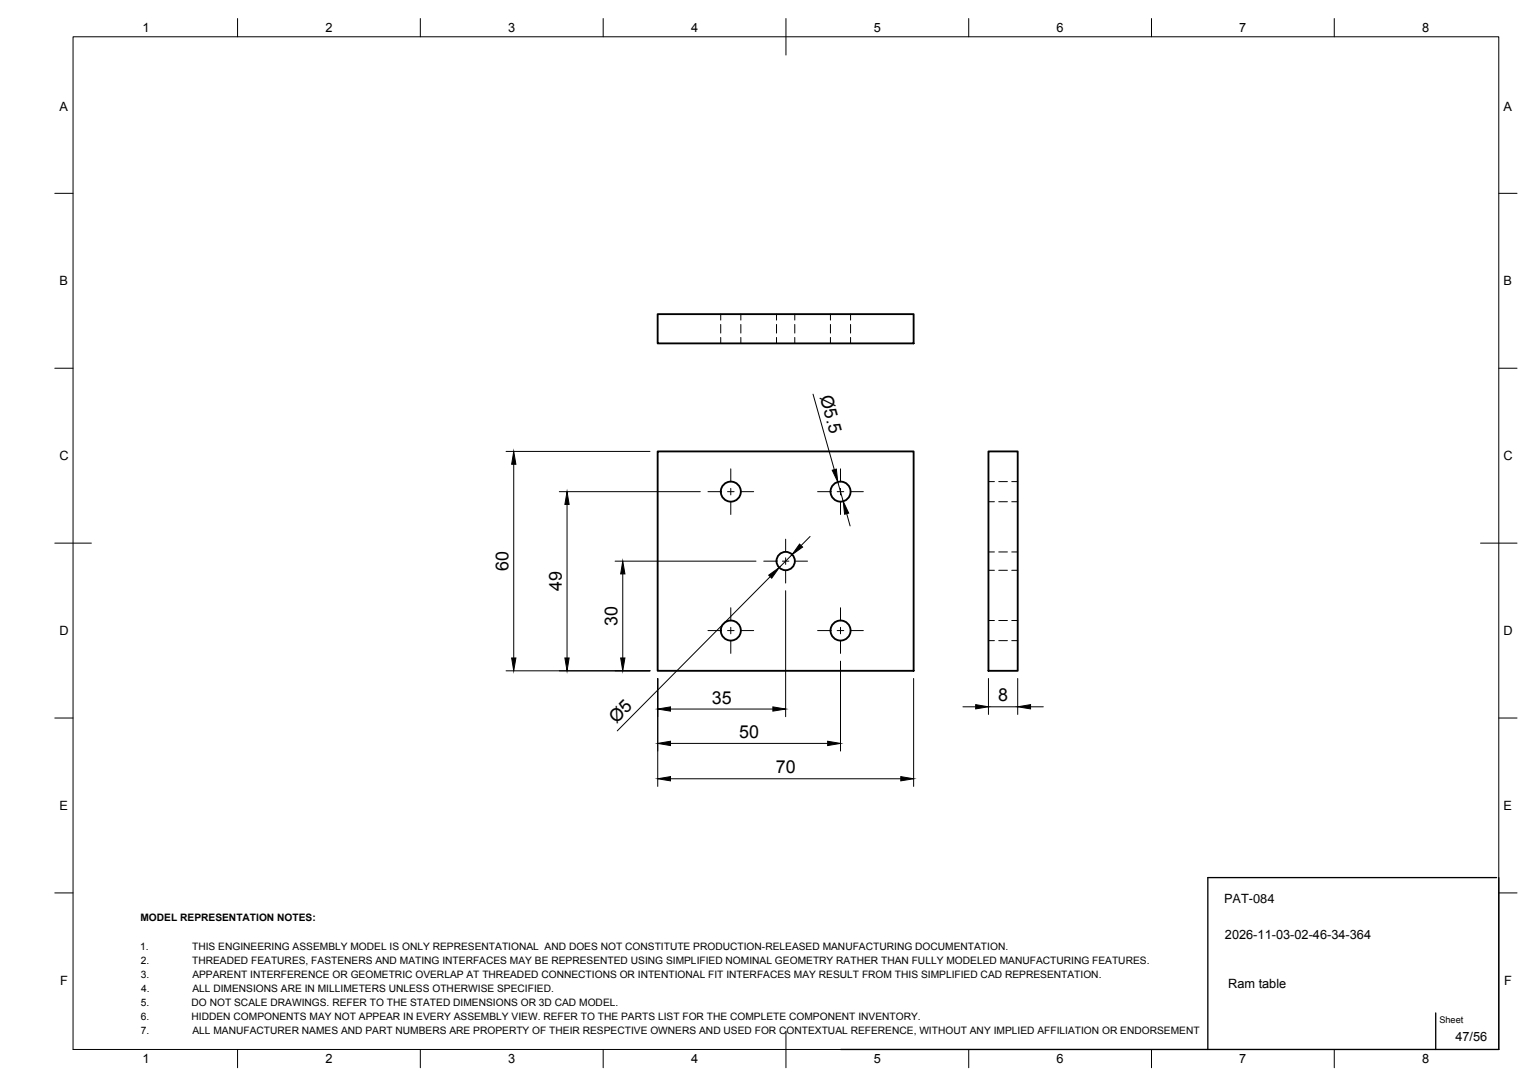
ISO-10303-21;
HEADER;
/* Generated by software containing ST-Developer
 * from STEP Tools, Inc. (www.steptools.com) 
 */

FILE_DESCRIPTION(
/* description */ ('Quick-return (Whitworth) mechanism'),
/* implementation_level */ '2;1');

FILE_NAME(
/* name */ 'Ram table.step',
/* time_stamp */ '2026-10-28T03:25:57-07:00',
/* author */ (''),
/* organization */ (''),
/* preprocessor_version */ 'ST-DEVELOPER v20.2',
/* originating_system */ 'Autodesk Translation Framework v15.17.0.0',
/* authorisation */ '');

FILE_SCHEMA (('AUTOMOTIVE_DESIGN { 1 0 10303 214 3 1 1 }'));
ENDSEC;

DATA;
#10=MECHANICAL_DESIGN_GEOMETRIC_PRESENTATION_REPRESENTATION('',(#532),#14878);
#436=SHAPE_REPRESENTATION_RELATIONSHIP('SRR','None',#15110,#480);
#480=ADVANCED_BREP_SHAPE_REPRESENTATION('',(#583),#14867);
#532=STYLED_ITEM('',(#15420),#583);
#583=MANIFOLD_SOLID_BREP('Body1',#7887);
#757=FACE_BOUND('',#2049,.T.);
#758=FACE_BOUND('',#2050,.T.);
#759=FACE_BOUND('',#2051,.T.);
#760=FACE_BOUND('',#2052,.T.);
#761=FACE_BOUND('',#2053,.T.);
#762=FACE_BOUND('',#2055,.T.);
#763=FACE_BOUND('',#2056,.T.);
#764=FACE_BOUND('',#2057,.T.);
#765=FACE_BOUND('',#2058,.T.);
#766=FACE_BOUND('',#2059,.T.);
#970=PLANE('',#9166);
#971=PLANE('',#9167);
#972=PLANE('',#9168);
#973=PLANE('',#9169);
#974=PLANE('',#9170);
#975=PLANE('',#9171);
#1407=FACE_OUTER_BOUND('',#2039,.T.);
#1408=FACE_OUTER_BOUND('',#2040,.T.);
#1409=FACE_OUTER_BOUND('',#2041,.T.);
#1410=FACE_OUTER_BOUND('',#2042,.T.);
#1411=FACE_OUTER_BOUND('',#2043,.T.);
#1412=FACE_OUTER_BOUND('',#2044,.T.);
#1413=FACE_OUTER_BOUND('',#2045,.T.);
#1414=FACE_OUTER_BOUND('',#2046,.T.);
#1415=FACE_OUTER_BOUND('',#2047,.T.);
#1416=FACE_OUTER_BOUND('',#2048,.T.);
#1417=FACE_OUTER_BOUND('',#2054,.T.);
#2039=EDGE_LOOP('',(#6736,#6737,#6738,#6739));
#2040=EDGE_LOOP('',(#6740,#6741,#6742,#6743));
#2041=EDGE_LOOP('',(#6744,#6745,#6746,#6747));
#2042=EDGE_LOOP('',(#6748,#6749,#6750,#6751));
#2043=EDGE_LOOP('',(#6752,#6753,#6754,#6755));
#2044=EDGE_LOOP('',(#6756,#6757,#6758,#6759));
#2045=EDGE_LOOP('',(#6760,#6761,#6762,#6763));
#2046=EDGE_LOOP('',(#6764,#6765,#6766,#6767));
#2047=EDGE_LOOP('',(#6768,#6769,#6770,#6771));
#2048=EDGE_LOOP('',(#6772,#6773,#6774,#6775));
#2049=EDGE_LOOP('',(#6776));
#2050=EDGE_LOOP('',(#6777));
#2051=EDGE_LOOP('',(#6778));
#2052=EDGE_LOOP('',(#6779));
#2053=EDGE_LOOP('',(#6780));
#2054=EDGE_LOOP('',(#6781,#6782,#6783,#6784));
#2055=EDGE_LOOP('',(#6785));
#2056=EDGE_LOOP('',(#6786));
#2057=EDGE_LOOP('',(#6787));
#2058=EDGE_LOOP('',(#6788));
#2059=EDGE_LOOP('',(#6789));
#2516=LINE('',#14196,#3039);
#2517=LINE('',#14202,#3040);
#2518=LINE('',#14208,#3041);
#2519=LINE('',#14214,#3042);
#2520=LINE('',#14220,#3043);
#2521=LINE('',#14225,#3044);
#2522=LINE('',#14227,#3045);
#2523=LINE('',#14229,#3046);
#2524=LINE('',#14230,#3047);
#2525=LINE('',#14233,#3048);
#2526=LINE('',#14235,#3049);
#2527=LINE('',#14236,#3050);
#2528=LINE('',#14239,#3051);
#2529=LINE('',#14241,#3052);
#2530=LINE('',#14242,#3053);
#2531=LINE('',#14244,#3054);
#2532=LINE('',#14245,#3055);
#3039=VECTOR('',#11281,0.25);
#3040=VECTOR('',#11288,0.275);
#3041=VECTOR('',#11295,0.275);
#3042=VECTOR('',#11302,0.275);
#3043=VECTOR('',#11309,0.275);
#3044=VECTOR('',#11314,1.);
#3045=VECTOR('',#11315,1.);
#3046=VECTOR('',#11316,1.);
#3047=VECTOR('',#11317,1.);
#3048=VECTOR('',#11320,1.);
#3049=VECTOR('',#11321,1.);
#3050=VECTOR('',#11322,1.);
#3051=VECTOR('',#11325,1.);
#3052=VECTOR('',#11326,1.);
#3053=VECTOR('',#11327,1.);
#3054=VECTOR('',#11330,1.);
#3055=VECTOR('',#11331,1.);
#3571=CIRCLE('',#9152,0.25);
#3572=CIRCLE('',#9153,0.25);
#3573=CIRCLE('',#9155,0.275);
#3574=CIRCLE('',#9156,0.275);
#3575=CIRCLE('',#9158,0.275);
#3576=CIRCLE('',#9159,0.275);
#3577=CIRCLE('',#9161,0.275);
#3578=CIRCLE('',#9162,0.275);
#3579=CIRCLE('',#9164,0.275);
#3580=CIRCLE('',#9165,0.275);
#4132=VERTEX_POINT('',#14193);
#4133=VERTEX_POINT('',#14195);
#4134=VERTEX_POINT('',#14199);
#4135=VERTEX_POINT('',#14201);
#4136=VERTEX_POINT('',#14205);
#4137=VERTEX_POINT('',#14207);
#4138=VERTEX_POINT('',#14211);
#4139=VERTEX_POINT('',#14213);
#4140=VERTEX_POINT('',#14217);
#4141=VERTEX_POINT('',#14219);
#4142=VERTEX_POINT('',#14223);
#4143=VERTEX_POINT('',#14224);
#4144=VERTEX_POINT('',#14226);
#4145=VERTEX_POINT('',#14228);
#4146=VERTEX_POINT('',#14232);
#4147=VERTEX_POINT('',#14234);
#4148=VERTEX_POINT('',#14238);
#4149=VERTEX_POINT('',#14240);
#5025=EDGE_CURVE('',#4132,#4132,#3571,.T.);
#5026=EDGE_CURVE('',#4132,#4133,#2516,.T.);
#5027=EDGE_CURVE('',#4133,#4133,#3572,.T.);
#5028=EDGE_CURVE('',#4134,#4134,#3573,.T.);
#5029=EDGE_CURVE('',#4134,#4135,#2517,.T.);
#5030=EDGE_CURVE('',#4135,#4135,#3574,.T.);
#5031=EDGE_CURVE('',#4136,#4136,#3575,.T.);
#5032=EDGE_CURVE('',#4136,#4137,#2518,.T.);
#5033=EDGE_CURVE('',#4137,#4137,#3576,.T.);
#5034=EDGE_CURVE('',#4138,#4138,#3577,.T.);
#5035=EDGE_CURVE('',#4138,#4139,#2519,.T.);
#5036=EDGE_CURVE('',#4139,#4139,#3578,.T.);
#5037=EDGE_CURVE('',#4140,#4140,#3579,.T.);
#5038=EDGE_CURVE('',#4140,#4141,#2520,.T.);
#5039=EDGE_CURVE('',#4141,#4141,#3580,.T.);
#5040=EDGE_CURVE('',#4142,#4143,#2521,.T.);
#5041=EDGE_CURVE('',#4143,#4144,#2522,.T.);
#5042=EDGE_CURVE('',#4145,#4144,#2523,.T.);
#5043=EDGE_CURVE('',#4142,#4145,#2524,.T.);
#5044=EDGE_CURVE('',#4146,#4142,#2525,.T.);
#5045=EDGE_CURVE('',#4147,#4145,#2526,.T.);
#5046=EDGE_CURVE('',#4146,#4147,#2527,.T.);
#5047=EDGE_CURVE('',#4148,#4146,#2528,.T.);
#5048=EDGE_CURVE('',#4149,#4147,#2529,.T.);
#5049=EDGE_CURVE('',#4148,#4149,#2530,.T.);
#5050=EDGE_CURVE('',#4143,#4148,#2531,.T.);
#5051=EDGE_CURVE('',#4144,#4149,#2532,.T.);
#6736=ORIENTED_EDGE('',*,*,#5025,.F.);
#6737=ORIENTED_EDGE('',*,*,#5026,.T.);
#6738=ORIENTED_EDGE('',*,*,#5027,.F.);
#6739=ORIENTED_EDGE('',*,*,#5026,.F.);
#6740=ORIENTED_EDGE('',*,*,#5028,.F.);
#6741=ORIENTED_EDGE('',*,*,#5029,.T.);
#6742=ORIENTED_EDGE('',*,*,#5030,.F.);
#6743=ORIENTED_EDGE('',*,*,#5029,.F.);
#6744=ORIENTED_EDGE('',*,*,#5031,.F.);
#6745=ORIENTED_EDGE('',*,*,#5032,.T.);
#6746=ORIENTED_EDGE('',*,*,#5033,.F.);
#6747=ORIENTED_EDGE('',*,*,#5032,.F.);
#6748=ORIENTED_EDGE('',*,*,#5034,.F.);
#6749=ORIENTED_EDGE('',*,*,#5035,.T.);
#6750=ORIENTED_EDGE('',*,*,#5036,.F.);
#6751=ORIENTED_EDGE('',*,*,#5035,.F.);
#6752=ORIENTED_EDGE('',*,*,#5037,.F.);
#6753=ORIENTED_EDGE('',*,*,#5038,.T.);
#6754=ORIENTED_EDGE('',*,*,#5039,.F.);
#6755=ORIENTED_EDGE('',*,*,#5038,.F.);
#6756=ORIENTED_EDGE('',*,*,#5040,.T.);
#6757=ORIENTED_EDGE('',*,*,#5041,.T.);
#6758=ORIENTED_EDGE('',*,*,#5042,.F.);
#6759=ORIENTED_EDGE('',*,*,#5043,.F.);
#6760=ORIENTED_EDGE('',*,*,#5044,.T.);
#6761=ORIENTED_EDGE('',*,*,#5043,.T.);
#6762=ORIENTED_EDGE('',*,*,#5045,.F.);
#6763=ORIENTED_EDGE('',*,*,#5046,.F.);
#6764=ORIENTED_EDGE('',*,*,#5047,.T.);
#6765=ORIENTED_EDGE('',*,*,#5046,.T.);
#6766=ORIENTED_EDGE('',*,*,#5048,.F.);
#6767=ORIENTED_EDGE('',*,*,#5049,.F.);
#6768=ORIENTED_EDGE('',*,*,#5050,.T.);
#6769=ORIENTED_EDGE('',*,*,#5049,.T.);
#6770=ORIENTED_EDGE('',*,*,#5051,.F.);
#6771=ORIENTED_EDGE('',*,*,#5041,.F.);
#6772=ORIENTED_EDGE('',*,*,#5051,.T.);
#6773=ORIENTED_EDGE('',*,*,#5048,.T.);
#6774=ORIENTED_EDGE('',*,*,#5045,.T.);
#6775=ORIENTED_EDGE('',*,*,#5042,.T.);
#6776=ORIENTED_EDGE('',*,*,#5027,.T.);
#6777=ORIENTED_EDGE('',*,*,#5030,.T.);
#6778=ORIENTED_EDGE('',*,*,#5033,.T.);
#6779=ORIENTED_EDGE('',*,*,#5036,.T.);
#6780=ORIENTED_EDGE('',*,*,#5039,.T.);
#6781=ORIENTED_EDGE('',*,*,#5050,.F.);
#6782=ORIENTED_EDGE('',*,*,#5040,.F.);
#6783=ORIENTED_EDGE('',*,*,#5044,.F.);
#6784=ORIENTED_EDGE('',*,*,#5047,.F.);
#6785=ORIENTED_EDGE('',*,*,#5025,.T.);
#6786=ORIENTED_EDGE('',*,*,#5028,.T.);
#6787=ORIENTED_EDGE('',*,*,#5031,.T.);
#6788=ORIENTED_EDGE('',*,*,#5034,.T.);
#6789=ORIENTED_EDGE('',*,*,#5037,.T.);
#7355=CYLINDRICAL_SURFACE('',#9151,0.25);
#7356=CYLINDRICAL_SURFACE('',#9154,0.275);
#7357=CYLINDRICAL_SURFACE('',#9157,0.275);
#7358=CYLINDRICAL_SURFACE('',#9160,0.275);
#7359=CYLINDRICAL_SURFACE('',#9163,0.275);
#7738=ADVANCED_FACE('',(#1407),#7355,.F.);
#7739=ADVANCED_FACE('',(#1408),#7356,.F.);
#7740=ADVANCED_FACE('',(#1409),#7357,.F.);
#7741=ADVANCED_FACE('',(#1410),#7358,.F.);
#7742=ADVANCED_FACE('',(#1411),#7359,.F.);
#7743=ADVANCED_FACE('',(#1412),#970,.T.);
#7744=ADVANCED_FACE('',(#1413),#971,.T.);
#7745=ADVANCED_FACE('',(#1414),#972,.T.);
#7746=ADVANCED_FACE('',(#1415),#973,.T.);
#7747=ADVANCED_FACE('',(#1416,#757,#758,#759,#760,#761),#974,.T.);
#7748=ADVANCED_FACE('',(#1417,#762,#763,#764,#765,#766),#975,.F.);
#7887=CLOSED_SHELL('',(#7738,#7739,#7740,#7741,#7742,#7743,#7744,#7745,
#7746,#7747,#7748));
#9150=AXIS2_PLACEMENT_3D('',#14191,#11275,#11276);
#9151=AXIS2_PLACEMENT_3D('',#14192,#11277,#11278);
#9152=AXIS2_PLACEMENT_3D('',#14194,#11279,#11280);
#9153=AXIS2_PLACEMENT_3D('',#14197,#11282,#11283);
#9154=AXIS2_PLACEMENT_3D('',#14198,#11284,#11285);
#9155=AXIS2_PLACEMENT_3D('',#14200,#11286,#11287);
#9156=AXIS2_PLACEMENT_3D('',#14203,#11289,#11290);
#9157=AXIS2_PLACEMENT_3D('',#14204,#11291,#11292);
#9158=AXIS2_PLACEMENT_3D('',#14206,#11293,#11294);
#9159=AXIS2_PLACEMENT_3D('',#14209,#11296,#11297);
#9160=AXIS2_PLACEMENT_3D('',#14210,#11298,#11299);
#9161=AXIS2_PLACEMENT_3D('',#14212,#11300,#11301);
#9162=AXIS2_PLACEMENT_3D('',#14215,#11303,#11304);
#9163=AXIS2_PLACEMENT_3D('',#14216,#11305,#11306);
#9164=AXIS2_PLACEMENT_3D('',#14218,#11307,#11308);
#9165=AXIS2_PLACEMENT_3D('',#14221,#11310,#11311);
#9166=AXIS2_PLACEMENT_3D('',#14222,#11312,#11313);
#9167=AXIS2_PLACEMENT_3D('',#14231,#11318,#11319);
#9168=AXIS2_PLACEMENT_3D('',#14237,#11323,#11324);
#9169=AXIS2_PLACEMENT_3D('',#14243,#11328,#11329);
#9170=AXIS2_PLACEMENT_3D('',#14246,#11332,#11333);
#9171=AXIS2_PLACEMENT_3D('',#14247,#11334,#11335);
#11275=DIRECTION('axis',(0.,0.,1.));
#11276=DIRECTION('refdir',(1.,0.,0.));
#11277=DIRECTION('center_axis',(0.,0.,1.));
#11278=DIRECTION('ref_axis',(1.,0.,0.));
#11279=DIRECTION('center_axis',(0.,0.,1.));
#11280=DIRECTION('ref_axis',(1.,0.,0.));
#11281=DIRECTION('',(0.,0.,1.));
#11282=DIRECTION('center_axis',(0.,0.,-1.));
#11283=DIRECTION('ref_axis',(1.,0.,0.));
#11284=DIRECTION('center_axis',(0.,0.,1.));
#11285=DIRECTION('ref_axis',(1.,0.,0.));
#11286=DIRECTION('center_axis',(0.,0.,1.));
#11287=DIRECTION('ref_axis',(1.,0.,0.));
#11288=DIRECTION('',(0.,0.,1.));
#11289=DIRECTION('center_axis',(0.,0.,-1.));
#11290=DIRECTION('ref_axis',(1.,0.,0.));
#11291=DIRECTION('center_axis',(0.,0.,1.));
#11292=DIRECTION('ref_axis',(1.,0.,0.));
#11293=DIRECTION('center_axis',(0.,0.,1.));
#11294=DIRECTION('ref_axis',(1.,0.,0.));
#11295=DIRECTION('',(0.,0.,1.));
#11296=DIRECTION('center_axis',(0.,0.,-1.));
#11297=DIRECTION('ref_axis',(1.,0.,0.));
#11298=DIRECTION('center_axis',(0.,0.,1.));
#11299=DIRECTION('ref_axis',(1.,0.,0.));
#11300=DIRECTION('center_axis',(0.,0.,1.));
#11301=DIRECTION('ref_axis',(1.,0.,0.));
#11302=DIRECTION('',(0.,0.,1.));
#11303=DIRECTION('center_axis',(0.,0.,-1.));
#11304=DIRECTION('ref_axis',(1.,0.,0.));
#11305=DIRECTION('center_axis',(0.,0.,1.));
#11306=DIRECTION('ref_axis',(1.,0.,0.));
#11307=DIRECTION('center_axis',(0.,0.,1.));
#11308=DIRECTION('ref_axis',(1.,0.,0.));
#11309=DIRECTION('',(0.,0.,1.));
#11310=DIRECTION('center_axis',(0.,0.,-1.));
#11311=DIRECTION('ref_axis',(1.,0.,0.));
#11312=DIRECTION('center_axis',(0.,1.,0.));
#11313=DIRECTION('ref_axis',(-1.,0.,0.));
#11314=DIRECTION('',(-1.,0.,0.));
#11315=DIRECTION('',(0.,0.,1.));
#11316=DIRECTION('',(-1.,0.,0.));
#11317=DIRECTION('',(0.,0.,1.));
#11318=DIRECTION('center_axis',(1.,0.,0.));
#11319=DIRECTION('ref_axis',(0.,1.,0.));
#11320=DIRECTION('',(0.,1.,0.));
#11321=DIRECTION('',(0.,1.,0.));
#11322=DIRECTION('',(0.,0.,1.));
#11323=DIRECTION('center_axis',(0.,-1.,0.));
#11324=DIRECTION('ref_axis',(1.,0.,0.));
#11325=DIRECTION('',(1.,0.,0.));
#11326=DIRECTION('',(1.,0.,0.));
#11327=DIRECTION('',(0.,0.,1.));
#11328=DIRECTION('center_axis',(-1.,0.,0.));
#11329=DIRECTION('ref_axis',(0.,-1.,0.));
#11330=DIRECTION('',(0.,-1.,0.));
#11331=DIRECTION('',(0.,-1.,0.));
#11332=DIRECTION('center_axis',(0.,0.,1.));
#11333=DIRECTION('ref_axis',(1.,0.,0.));
#11334=DIRECTION('center_axis',(0.,0.,1.));
#11335=DIRECTION('ref_axis',(1.,0.,0.));
#14191=CARTESIAN_POINT('',(0.,0.,0.));
#14192=CARTESIAN_POINT('Origin',(9.16515138991168,16.,3.3));
#14193=CARTESIAN_POINT('',(8.91515138991168,16.,3.4));
#14194=CARTESIAN_POINT('Origin',(9.16515138991168,16.,3.4));
#14195=CARTESIAN_POINT('',(8.91515138991168,16.,4.2));
#14196=CARTESIAN_POINT('',(8.91515138991168,16.,3.3));
#14197=CARTESIAN_POINT('Origin',(9.16515138991168,16.,4.2));
#14198=CARTESIAN_POINT('Origin',(10.6651513899117,14.1,3.3));
#14199=CARTESIAN_POINT('',(10.3901513899117,14.1,3.4));
#14200=CARTESIAN_POINT('Origin',(10.6651513899117,14.1,3.4));
#14201=CARTESIAN_POINT('',(10.3901513899117,14.1,4.2));
#14202=CARTESIAN_POINT('',(10.3901513899117,14.1,3.3));
#14203=CARTESIAN_POINT('Origin',(10.6651513899117,14.1,4.2));
#14204=CARTESIAN_POINT('Origin',(7.66515138991168,17.9,3.3));
#14205=CARTESIAN_POINT('',(7.39015138991168,17.9,3.4));
#14206=CARTESIAN_POINT('Origin',(7.66515138991168,17.9,3.4));
#14207=CARTESIAN_POINT('',(7.39015138991168,17.9,4.2));
#14208=CARTESIAN_POINT('',(7.39015138991168,17.9,3.3));
#14209=CARTESIAN_POINT('Origin',(7.66515138991168,17.9,4.2));
#14210=CARTESIAN_POINT('Origin',(7.66515138991168,14.1,3.3));
#14211=CARTESIAN_POINT('',(7.39015138991168,14.1,3.4));
#14212=CARTESIAN_POINT('Origin',(7.66515138991168,14.1,3.4));
#14213=CARTESIAN_POINT('',(7.39015138991168,14.1,4.2));
#14214=CARTESIAN_POINT('',(7.39015138991168,14.1,3.3));
#14215=CARTESIAN_POINT('Origin',(7.66515138991168,14.1,4.2));
#14216=CARTESIAN_POINT('Origin',(10.6651513899117,17.9,3.3));
#14217=CARTESIAN_POINT('',(10.3901513899117,17.9,3.4));
#14218=CARTESIAN_POINT('Origin',(10.6651513899117,17.9,3.4));
#14219=CARTESIAN_POINT('',(10.3901513899117,17.9,4.2));
#14220=CARTESIAN_POINT('',(10.3901513899117,17.9,3.3));
#14221=CARTESIAN_POINT('Origin',(10.6651513899117,17.9,4.2));
#14222=CARTESIAN_POINT('Origin',(12.6651513899117,19.,3.4));
#14223=CARTESIAN_POINT('',(12.6651513899117,19.,3.4));
#14224=CARTESIAN_POINT('',(5.66515138991168,19.,3.4));
#14225=CARTESIAN_POINT('',(12.6651513899117,19.,3.4));
#14226=CARTESIAN_POINT('',(5.66515138991168,19.,4.2));
#14227=CARTESIAN_POINT('',(5.66515138991168,19.,3.4));
#14228=CARTESIAN_POINT('',(12.6651513899117,19.,4.2));
#14229=CARTESIAN_POINT('',(12.6651513899117,19.,4.2));
#14230=CARTESIAN_POINT('',(12.6651513899117,19.,3.4));
#14231=CARTESIAN_POINT('Origin',(12.6651513899117,13.,3.4));
#14232=CARTESIAN_POINT('',(12.6651513899117,13.,3.4));
#14233=CARTESIAN_POINT('',(12.6651513899117,13.,3.4));
#14234=CARTESIAN_POINT('',(12.6651513899117,13.,4.2));
#14235=CARTESIAN_POINT('',(12.6651513899117,13.,4.2));
#14236=CARTESIAN_POINT('',(12.6651513899117,13.,3.4));
#14237=CARTESIAN_POINT('Origin',(5.66515138991168,13.,3.4));
#14238=CARTESIAN_POINT('',(5.66515138991168,13.,3.4));
#14239=CARTESIAN_POINT('',(5.66515138991168,13.,3.4));
#14240=CARTESIAN_POINT('',(5.66515138991168,13.,4.2));
#14241=CARTESIAN_POINT('',(5.66515138991168,13.,4.2));
#14242=CARTESIAN_POINT('',(5.66515138991168,13.,3.4));
#14243=CARTESIAN_POINT('Origin',(5.66515138991168,19.,3.4));
#14244=CARTESIAN_POINT('',(5.66515138991168,19.,3.4));
#14245=CARTESIAN_POINT('',(5.66515138991168,19.,4.2));
#14246=CARTESIAN_POINT('Origin',(9.16515138991168,16.,4.2));
#14247=CARTESIAN_POINT('Origin',(9.16515138991168,16.,3.4));
#14813=UNCERTAINTY_MEASURE_WITH_UNIT(LENGTH_MEASURE(0.001),#14879,
'DISTANCE_ACCURACY_VALUE',
'Maximum model space distance between geometric entities at asserted c
onnectivities');
#14824=UNCERTAINTY_MEASURE_WITH_UNIT(LENGTH_MEASURE(0.001),#14879,
'DISTANCE_ACCURACY_VALUE',
'Maximum model space distance between geometric entities at asserted c
onnectivities');
#14867=(
GEOMETRIC_REPRESENTATION_CONTEXT(3)
GLOBAL_UNCERTAINTY_ASSIGNED_CONTEXT((#14813))
GLOBAL_UNIT_ASSIGNED_CONTEXT((#14879,#14881,#14882))
REPRESENTATION_CONTEXT('','3D')
);
#14878=(
GEOMETRIC_REPRESENTATION_CONTEXT(3)
GLOBAL_UNCERTAINTY_ASSIGNED_CONTEXT((#14824))
GLOBAL_UNIT_ASSIGNED_CONTEXT((#14879,#14881,#14882))
REPRESENTATION_CONTEXT('','3D')
);
#14879=(
LENGTH_UNIT()
NAMED_UNIT(*)
SI_UNIT(.CENTI.,.METRE.)
);
#14881=(
NAMED_UNIT(*)
PLANE_ANGLE_UNIT()
SI_UNIT($,.RADIAN.)
);
#14882=(
NAMED_UNIT(*)
SI_UNIT($,.STERADIAN.)
SOLID_ANGLE_UNIT()
);
#14925=SHAPE_DEFINITION_REPRESENTATION(#14987,#15110);
#14987=PRODUCT_DEFINITION_SHAPE('',$,#15164);
#15110=SHAPE_REPRESENTATION('',(#9150),#14867);
#15121=PRODUCT_DEFINITION_CONTEXT('part definition',#15282,'design');
#15164=PRODUCT_DEFINITION('Ram table','Ram table',#15217,#15121);
#15217=PRODUCT_DEFINITION_FORMATION('',$,#15326);
#15282=APPLICATION_CONTEXT(
'Core Data for Automotive Mechanical Design Process');
#15283=PRODUCT_CONTEXT('part definition',#15282,'mechanical');
#15326=PRODUCT('Ram table','Ram table','Ram table',(#15283));
#15414=COLOUR_RGB('Off White',0.89,0.88,0.83);
#15415=FILL_AREA_STYLE_COLOUR('',#15414);
#15416=FILL_AREA_STYLE('',(#15415));
#15417=SURFACE_STYLE_FILL_AREA(#15416);
#15418=SURFACE_SIDE_STYLE('',(#15417));
#15419=SURFACE_STYLE_USAGE(.BOTH.,#15418);
#15420=PRESENTATION_STYLE_ASSIGNMENT((#15419));
ENDSEC;
END-ISO-10303-21;
